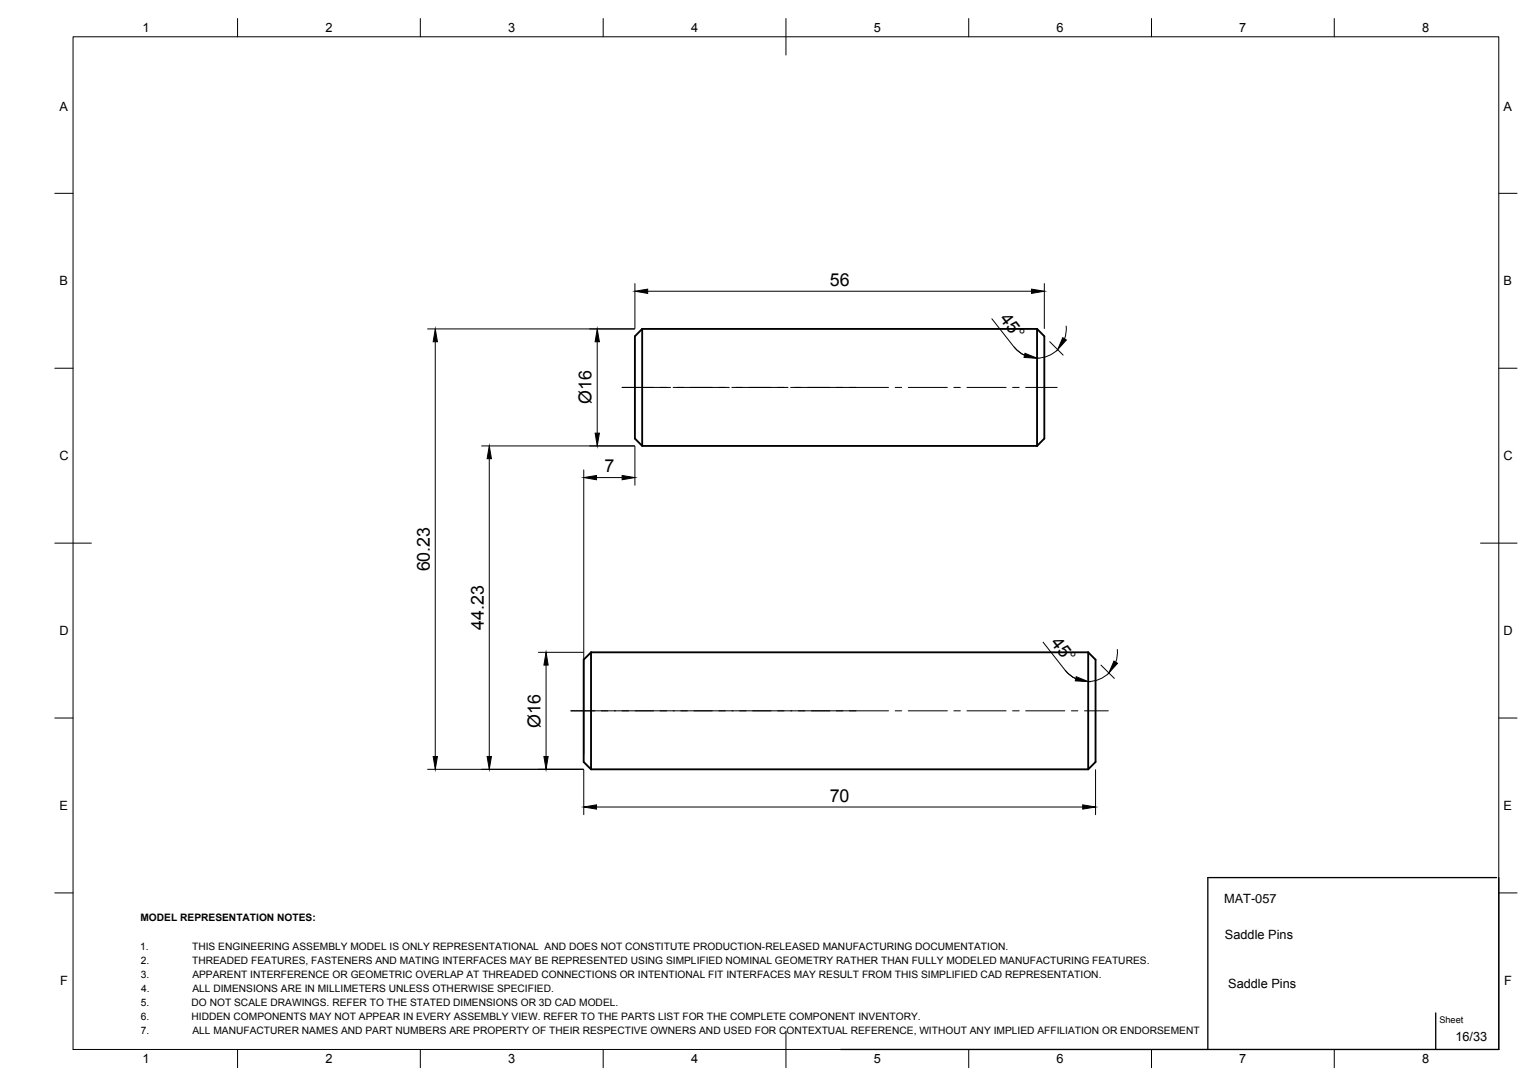
ISO-10303-21;
HEADER;
/* Generated by software containing ST-Developer
 * from STEP Tools, Inc. (www.steptools.com) 
 */

FILE_DESCRIPTION(
/* description */ ('STEP AP214', 'CAx-IF Rec.Pracs.---Representation and Presentation of Product Manufa
cturing Information (PMI)---4.0---2014-10-13'),
/* implementation_level */ '2;1');

FILE_NAME(
/* name */ 'Saddle Pins.step',
/* time_stamp */ '2026-10-28T23:34:22+01:00',
/* author */ (''),
/* organization */ (''),
/* preprocessor_version */ 'ST-DEVELOPER v20.2',
/* originating_system */ 'Autodesk Translation Framework v15.17.0.0',
/* authorisation */ '');

FILE_SCHEMA (('AP242_MANAGED_MODEL_BASED_3D_ENGINEERING_MIM_LF { 1 0 10303 442 2 1 4 }'));
ENDSEC;

DATA;
#10=MECHANICAL_DESIGN_GEOMETRIC_PRESENTATION_REPRESENTATION('',(#256,#257),#27807);
#211=SHAPE_REPRESENTATION_RELATIONSHIP('SRR','None',#27907,#233);
#233=ADVANCED_BREP_SHAPE_REPRESENTATION('',(#285,#286),#27787);
#256=STYLED_ITEM('',(#28063),#285);
#257=STYLED_ITEM('',(#28063),#286);
#285=MANIFOLD_SOLID_BREP('Body1',#12032);
#286=MANIFOLD_SOLID_BREP('Body2',#12033);
#578=PLANE('',#12953);
#579=PLANE('',#12954);
#580=PLANE('',#12963);
#581=PLANE('',#12964);
#1091=CYLINDRICAL_SURFACE('',#12952,8.00000000000001);
#1092=CYLINDRICAL_SURFACE('',#12962,8.);
#1541=FACE_OUTER_BOUND('',#2296,.T.);
#1542=FACE_OUTER_BOUND('',#2297,.T.);
#1543=FACE_OUTER_BOUND('',#2298,.T.);
#1544=FACE_OUTER_BOUND('',#2299,.T.);
#1545=FACE_OUTER_BOUND('',#2300,.T.);
#1546=FACE_OUTER_BOUND('',#2301,.T.);
#1547=FACE_OUTER_BOUND('',#2302,.T.);
#1548=FACE_OUTER_BOUND('',#2303,.T.);
#1549=FACE_OUTER_BOUND('',#2304,.T.);
#1550=FACE_OUTER_BOUND('',#2305,.T.);
#2296=EDGE_LOOP('',(#9389,#9390,#9391,#9392));
#2297=EDGE_LOOP('',(#9393,#9394,#9395,#9396,#9397));
#2298=EDGE_LOOP('',(#9398,#9399,#9400,#9401,#9402));
#2299=EDGE_LOOP('',(#9403));
#2300=EDGE_LOOP('',(#9404));
#2301=EDGE_LOOP('',(#9405,#9406,#9407,#9408));
#2302=EDGE_LOOP('',(#9409,#9410,#9411,#9412,#9413));
#2303=EDGE_LOOP('',(#9414,#9415,#9416,#9417,#9418));
#2304=EDGE_LOOP('',(#9419));
#2305=EDGE_LOOP('',(#9420));
#3136=LINE('',#19300,#3956);
#3137=LINE('',#19308,#3957);
#3138=LINE('',#19311,#3958);
#3139=LINE('',#19318,#3959);
#3140=LINE('',#19326,#3960);
#3141=LINE('',#19329,#3961);
#3956=VECTOR('',#15412,7.);
#3957=VECTOR('',#15421,8.00000000000001);
#3958=VECTOR('',#15426,8.00000000000001);
#3959=VECTOR('',#15435,7.);
#3960=VECTOR('',#15444,8.);
#3961=VECTOR('',#15449,8.);
#4713=CIRCLE('',#12946,8.00000000000001);
#4714=CIRCLE('',#12947,7.);
#4715=CIRCLE('',#12949,8.00000000000001);
#4716=CIRCLE('',#12950,8.00000000000001);
#4717=CIRCLE('',#12951,7.);
#4718=CIRCLE('',#12956,8.);
#4719=CIRCLE('',#12957,7.);
#4720=CIRCLE('',#12959,8.);
#4721=CIRCLE('',#12960,8.);
#4722=CIRCLE('',#12961,7.);
#5534=VERTEX_POINT('',#19297);
#5535=VERTEX_POINT('',#19299);
#5536=VERTEX_POINT('',#19303);
#5537=VERTEX_POINT('',#19304);
#5538=VERTEX_POINT('',#19307);
#5539=VERTEX_POINT('',#19315);
#5540=VERTEX_POINT('',#19317);
#5541=VERTEX_POINT('',#19321);
#5542=VERTEX_POINT('',#19322);
#5543=VERTEX_POINT('',#19325);
#6907=EDGE_CURVE('',#5534,#5534,#4713,.T.);
#6908=EDGE_CURVE('',#5534,#5535,#3136,.T.);
#6909=EDGE_CURVE('',#5535,#5535,#4714,.T.);
#6910=EDGE_CURVE('',#5536,#5537,#4715,.T.);
#6911=EDGE_CURVE('',#5537,#5536,#4716,.T.);
#6912=EDGE_CURVE('',#5537,#5538,#3137,.T.);
#6913=EDGE_CURVE('',#5538,#5538,#4717,.T.);
#6914=EDGE_CURVE('',#5536,#5534,#3138,.T.);
#6915=EDGE_CURVE('',#5539,#5539,#4718,.T.);
#6916=EDGE_CURVE('',#5539,#5540,#3139,.T.);
#6917=EDGE_CURVE('',#5540,#5540,#4719,.T.);
#6918=EDGE_CURVE('',#5541,#5542,#4720,.T.);
#6919=EDGE_CURVE('',#5542,#5541,#4721,.T.);
#6920=EDGE_CURVE('',#5542,#5543,#3140,.T.);
#6921=EDGE_CURVE('',#5543,#5543,#4722,.T.);
#6922=EDGE_CURVE('',#5541,#5539,#3141,.T.);
#9389=ORIENTED_EDGE('',*,*,#6907,.F.);
#9390=ORIENTED_EDGE('',*,*,#6908,.T.);
#9391=ORIENTED_EDGE('',*,*,#6909,.F.);
#9392=ORIENTED_EDGE('',*,*,#6908,.F.);
#9393=ORIENTED_EDGE('',*,*,#6910,.F.);
#9394=ORIENTED_EDGE('',*,*,#6911,.F.);
#9395=ORIENTED_EDGE('',*,*,#6912,.T.);
#9396=ORIENTED_EDGE('',*,*,#6913,.F.);
#9397=ORIENTED_EDGE('',*,*,#6912,.F.);
#9398=ORIENTED_EDGE('',*,*,#6910,.T.);
#9399=ORIENTED_EDGE('',*,*,#6911,.T.);
#9400=ORIENTED_EDGE('',*,*,#6914,.T.);
#9401=ORIENTED_EDGE('',*,*,#6907,.T.);
#9402=ORIENTED_EDGE('',*,*,#6914,.F.);
#9403=ORIENTED_EDGE('',*,*,#6909,.T.);
#9404=ORIENTED_EDGE('',*,*,#6913,.T.);
#9405=ORIENTED_EDGE('',*,*,#6915,.F.);
#9406=ORIENTED_EDGE('',*,*,#6916,.T.);
#9407=ORIENTED_EDGE('',*,*,#6917,.F.);
#9408=ORIENTED_EDGE('',*,*,#6916,.F.);
#9409=ORIENTED_EDGE('',*,*,#6918,.F.);
#9410=ORIENTED_EDGE('',*,*,#6919,.F.);
#9411=ORIENTED_EDGE('',*,*,#6920,.T.);
#9412=ORIENTED_EDGE('',*,*,#6921,.F.);
#9413=ORIENTED_EDGE('',*,*,#6920,.F.);
#9414=ORIENTED_EDGE('',*,*,#6918,.T.);
#9415=ORIENTED_EDGE('',*,*,#6919,.T.);
#9416=ORIENTED_EDGE('',*,*,#6922,.T.);
#9417=ORIENTED_EDGE('',*,*,#6915,.T.);
#9418=ORIENTED_EDGE('',*,*,#6922,.F.);
#9419=ORIENTED_EDGE('',*,*,#6917,.T.);
#9420=ORIENTED_EDGE('',*,*,#6921,.T.);
#11301=CONICAL_SURFACE('',#12945,7.,0.785398163397443);
#11302=CONICAL_SURFACE('',#12948,8.00000000000001,0.785398163397448);
#11303=CONICAL_SURFACE('',#12955,7.,0.785398163397445);
#11304=CONICAL_SURFACE('',#12958,8.,0.785398163397455);
#11623=ADVANCED_FACE('',(#1541),#11301,.T.);
#11624=ADVANCED_FACE('',(#1542),#11302,.T.);
#11625=ADVANCED_FACE('',(#1543),#1091,.T.);
#11626=ADVANCED_FACE('',(#1544),#578,.T.);
#11627=ADVANCED_FACE('',(#1545),#579,.F.);
#11628=ADVANCED_FACE('',(#1546),#11303,.T.);
#11629=ADVANCED_FACE('',(#1547),#11304,.T.);
#11630=ADVANCED_FACE('',(#1548),#1092,.T.);
#11631=ADVANCED_FACE('',(#1549),#580,.T.);
#11632=ADVANCED_FACE('',(#1550),#581,.F.);
#12032=CLOSED_SHELL('',(#11623,#11624,#11625,#11626,#11627));
#12033=CLOSED_SHELL('',(#11628,#11629,#11630,#11631,#11632));
#12944=AXIS2_PLACEMENT_3D('',#19295,#15406,#15407);
#12945=AXIS2_PLACEMENT_3D('',#19296,#15408,#15409);
#12946=AXIS2_PLACEMENT_3D('',#19298,#15410,#15411);
#12947=AXIS2_PLACEMENT_3D('',#19301,#15413,#15414);
#12948=AXIS2_PLACEMENT_3D('',#19302,#15415,#15416);
#12949=AXIS2_PLACEMENT_3D('',#19305,#15417,#15418);
#12950=AXIS2_PLACEMENT_3D('',#19306,#15419,#15420);
#12951=AXIS2_PLACEMENT_3D('',#19309,#15422,#15423);
#12952=AXIS2_PLACEMENT_3D('',#19310,#15424,#15425);
#12953=AXIS2_PLACEMENT_3D('',#19312,#15427,#15428);
#12954=AXIS2_PLACEMENT_3D('',#19313,#15429,#15430);
#12955=AXIS2_PLACEMENT_3D('',#19314,#15431,#15432);
#12956=AXIS2_PLACEMENT_3D('',#19316,#15433,#15434);
#12957=AXIS2_PLACEMENT_3D('',#19319,#15436,#15437);
#12958=AXIS2_PLACEMENT_3D('',#19320,#15438,#15439);
#12959=AXIS2_PLACEMENT_3D('',#19323,#15440,#15441);
#12960=AXIS2_PLACEMENT_3D('',#19324,#15442,#15443);
#12961=AXIS2_PLACEMENT_3D('',#19327,#15445,#15446);
#12962=AXIS2_PLACEMENT_3D('',#19328,#15447,#15448);
#12963=AXIS2_PLACEMENT_3D('',#19330,#15450,#15451);
#12964=AXIS2_PLACEMENT_3D('',#19331,#15452,#15453);
#15406=DIRECTION('axis',(0.,0.,1.));
#15407=DIRECTION('refdir',(1.,0.,0.));
#15408=DIRECTION('center_axis',(0.,0.,-1.));
#15409=DIRECTION('ref_axis',(-0.99771030462832,0.067632448118233,0.));
#15410=DIRECTION('center_axis',(0.,0.,-1.));
#15411=DIRECTION('ref_axis',(0.99771030462832,-0.0676324481182314,0.));
#15412=DIRECTION('',(-0.705487722062377,0.0478233626926498,0.707106781186551));
#15413=DIRECTION('center_axis',(0.,0.,1.));
#15414=DIRECTION('ref_axis',(0.99771030462832,-0.067632448118233,0.));
#15415=DIRECTION('center_axis',(0.,0.,1.));
#15416=DIRECTION('ref_axis',(0.99771030462832,-0.0676324481182314,0.));
#15417=DIRECTION('center_axis',(0.,0.,1.));
#15418=DIRECTION('ref_axis',(0.99771030462832,-0.0676324481182314,0.));
#15419=DIRECTION('center_axis',(0.,0.,1.));
#15420=DIRECTION('ref_axis',(0.99771030462832,-0.0676324481182314,0.));
#15421=DIRECTION('',(0.705487722062381,-0.0478233626926487,-0.707106781186547));
#15422=DIRECTION('center_axis',(0.,0.,-1.));
#15423=DIRECTION('ref_axis',(0.99771030462832,-0.0676324481182291,0.));
#15424=DIRECTION('center_axis',(0.,0.,-1.));
#15425=DIRECTION('ref_axis',(-0.99771030462832,0.0676324481182314,0.));
#15426=DIRECTION('',(0.,0.,1.));
#15427=DIRECTION('center_axis',(0.,0.,1.));
#15428=DIRECTION('ref_axis',(0.99771030462832,-0.0676324481182317,0.));
#15429=DIRECTION('center_axis',(0.,0.,1.));
#15430=DIRECTION('ref_axis',(0.99771030462832,-0.0676324481182317,0.));
#15431=DIRECTION('center_axis',(0.,0.,-1.));
#15432=DIRECTION('ref_axis',(-0.999999893830928,0.00046080162076951,0.));
#15433=DIRECTION('center_axis',(0.,0.,-1.));
#15434=DIRECTION('ref_axis',(0.999999893830927,-0.000460801620770501,0.));
#15435=DIRECTION('',(-0.707106706113674,0.000325835950827958,0.70710678118655));
#15436=DIRECTION('center_axis',(0.,0.,1.));
#15437=DIRECTION('ref_axis',(0.999999893830928,-0.00046080162076951,0.));
#15438=DIRECTION('center_axis',(0.,0.,1.));
#15439=DIRECTION('ref_axis',(0.999999893830927,-0.000460801620770501,0.));
#15440=DIRECTION('center_axis',(0.,0.,1.));
#15441=DIRECTION('ref_axis',(0.999999893830927,-0.000460801620770501,0.));
#15442=DIRECTION('center_axis',(0.,0.,1.));
#15443=DIRECTION('ref_axis',(0.999999893830927,-0.000460801620770501,0.));
#15444=DIRECTION('',(0.707106706113681,-0.000325835950828489,-0.707106781186542));
#15445=DIRECTION('center_axis',(0.,0.,-1.));
#15446=DIRECTION('ref_axis',(0.999999893830928,-0.00046080162076951,0.));
#15447=DIRECTION('center_axis',(0.,0.,-1.));
#15448=DIRECTION('ref_axis',(-0.999999893830927,0.000460801620770501,0.));
#15449=DIRECTION('',(0.,0.,1.));
#15450=DIRECTION('center_axis',(0.,0.,1.));
#15451=DIRECTION('ref_axis',(0.999999893830928,-0.00046080162077021,0.));
#15452=DIRECTION('center_axis',(0.,0.,1.));
#15453=DIRECTION('ref_axis',(0.999999893830928,-0.00046080162077021,0.));
#19295=CARTESIAN_POINT('',(0.,0.,0.));
#19296=CARTESIAN_POINT('Origin',(-232.939627118415,176.278148255596,281.073593133703));
#19297=CARTESIAN_POINT('',(-224.957944681388,175.73708867065,280.073593133703));
#19298=CARTESIAN_POINT('Origin',(-232.939627118415,176.278148255596,280.073593133703));
#19299=CARTESIAN_POINT('',(-225.955654986017,175.804721118769,281.073593133703));
#19300=CARTESIAN_POINT('',(-225.955654986017,175.804721118769,281.073593133703));
#19301=CARTESIAN_POINT('Origin',(-232.939627118415,176.278148255596,281.073593133703));
#19302=CARTESIAN_POINT('Origin',(-232.939627118415,176.278148255596,226.073593133703));
#19303=CARTESIAN_POINT('',(-224.957944681388,175.73708867065,226.073593133703));
#19304=CARTESIAN_POINT('',(-240.921309555442,176.819207840542,226.073593133703));
#19305=CARTESIAN_POINT('Origin',(-232.939627118415,176.278148255596,226.073593133703));
#19306=CARTESIAN_POINT('Origin',(-232.939627118415,176.278148255596,226.073593133703));
#19307=CARTESIAN_POINT('',(-239.923599250813,176.751575392424,225.073593133703));
#19308=CARTESIAN_POINT('',(-240.921309555442,176.819207840542,226.073593133703));
#19309=CARTESIAN_POINT('Origin',(-232.939627118415,176.278148255596,225.073593133703));
#19310=CARTESIAN_POINT('Origin',(-232.939627118415,176.278148255596,281.073593133703));
#19311=CARTESIAN_POINT('',(-224.957944681388,175.73708867065,281.073593133703));
#19312=CARTESIAN_POINT('Origin',(-232.939627118415,176.278148255596,281.073593133703));
#19313=CARTESIAN_POINT('Origin',(-232.939627118415,176.278148255596,225.073593133703));
#19314=CARTESIAN_POINT('Origin',(-256.26210404747,132.050757761767,288.073593133703));
#19315=CARTESIAN_POINT('',(-248.262104896823,132.047071348801,287.073593133703));
#19316=CARTESIAN_POINT('Origin',(-256.26210404747,132.050757761767,287.073593133703));
#19317=CARTESIAN_POINT('',(-249.262104790654,132.047532150421,288.073593133703));
#19318=CARTESIAN_POINT('',(-249.262104790654,132.047532150421,288.073593133703));
#19319=CARTESIAN_POINT('Origin',(-256.26210404747,132.050757761767,288.073593133703));
#19320=CARTESIAN_POINT('Origin',(-256.26210404747,132.050757761767,219.073593133703));
#19321=CARTESIAN_POINT('',(-248.262104896823,132.047071348801,219.073593133703));
#19322=CARTESIAN_POINT('',(-264.262103198118,132.054444174733,219.073593133703));
#19323=CARTESIAN_POINT('Origin',(-256.26210404747,132.050757761767,219.073593133703));
#19324=CARTESIAN_POINT('Origin',(-256.26210404747,132.050757761767,219.073593133703));
#19325=CARTESIAN_POINT('',(-263.262103304287,132.053983373112,218.073593133703));
#19326=CARTESIAN_POINT('',(-264.262103198118,132.054444174733,219.073593133703));
#19327=CARTESIAN_POINT('Origin',(-256.26210404747,132.050757761767,218.073593133703));
#19328=CARTESIAN_POINT('Origin',(-256.26210404747,132.050757761767,288.073593133703));
#19329=CARTESIAN_POINT('',(-248.262104896823,132.047071348801,288.073593133703));
#19330=CARTESIAN_POINT('Origin',(-256.26210404747,132.050757761767,288.073593133703));
#19331=CARTESIAN_POINT('Origin',(-256.26210404747,132.050757761767,218.073593133703));
#27758=UNCERTAINTY_MEASURE_WITH_UNIT(LENGTH_MEASURE(0.01),#27808,
'DISTANCE_ACCURACY_VALUE',
'Maximum model space distance between geometric entities at asserted c
onnectivities');
#27778=UNCERTAINTY_MEASURE_WITH_UNIT(LENGTH_MEASURE(0.01),#27808,
'DISTANCE_ACCURACY_VALUE',
'Maximum model space distance between geometric entities at asserted c
onnectivities');
#27787=(
GEOMETRIC_REPRESENTATION_CONTEXT(3)
GLOBAL_UNCERTAINTY_ASSIGNED_CONTEXT((#27758))
GLOBAL_UNIT_ASSIGNED_CONTEXT((#27808,#27810,#27811))
REPRESENTATION_CONTEXT('','3D')
);
#27807=(
GEOMETRIC_REPRESENTATION_CONTEXT(3)
GLOBAL_UNCERTAINTY_ASSIGNED_CONTEXT((#27778))
GLOBAL_UNIT_ASSIGNED_CONTEXT((#27808,#27810,#27811))
REPRESENTATION_CONTEXT('','3D')
);
#27808=(
LENGTH_UNIT()
NAMED_UNIT(*)
SI_UNIT(.MILLI.,.METRE.)
);
#27810=(
NAMED_UNIT(*)
PLANE_ANGLE_UNIT()
SI_UNIT($,.RADIAN.)
);
#27811=(
NAMED_UNIT(*)
SI_UNIT($,.STERADIAN.)
SOLID_ANGLE_UNIT()
);
#27820=SHAPE_DEFINITION_REPRESENTATION(#27850,#27907);
#27850=PRODUCT_DEFINITION_SHAPE('',$,#27936);
#27907=SHAPE_REPRESENTATION('',(#12944),#27787);
#27927=PRODUCT_DEFINITION_CONTEXT('part definition',#28013,'design');
#27936=PRODUCT_DEFINITION('Saddle Pins','Saddle Pins',#27964,#27927);
#27964=PRODUCT_DEFINITION_FORMATION('',$,#28023);
#28013=APPLICATION_CONTEXT('Managed model based 3d engineering');
#28014=PRODUCT_CONTEXT('part definition',#28013,'mechanical');
#28023=PRODUCT('Saddle Pins','Saddle Pins',$,(#28014));
#28057=COLOUR_RGB('Light Blue',0.38,0.62,0.78);
#28058=FILL_AREA_STYLE_COLOUR('',#28057);
#28059=FILL_AREA_STYLE('',(#28058));
#28060=SURFACE_STYLE_FILL_AREA(#28059);
#28061=SURFACE_SIDE_STYLE('',(#28060));
#28062=SURFACE_STYLE_USAGE(.BOTH.,#28061);
#28063=PRESENTATION_STYLE_ASSIGNMENT((#28062));
ENDSEC;
END-ISO-10303-21;
